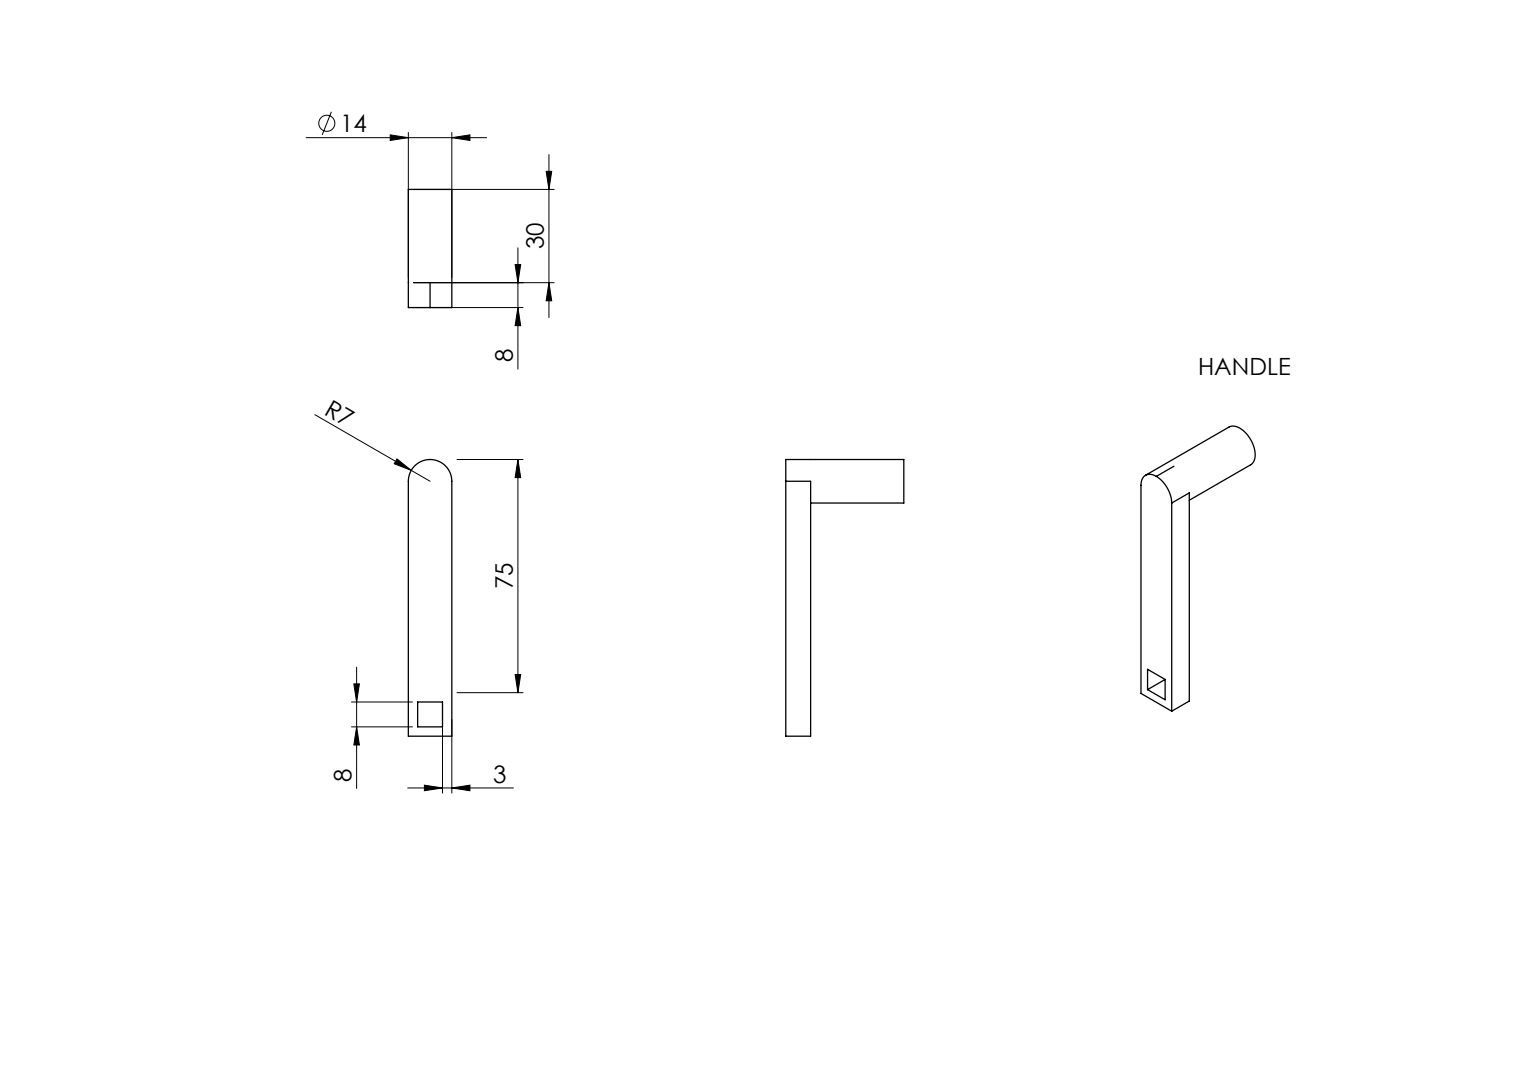
ISO-10303-21;
HEADER;
FILE_DESCRIPTION (('STEP AP214'),
    '1' );
FILE_NAME ('handle.step',
    '2026-10-27T17:01:19',
    ( '' ),
    ( '' ),
    'SwSTEP 2.0',
    'SolidWorks 2026',
    '' );
FILE_SCHEMA (( 'AUTOMOTIVE_DESIGN' ));
ENDSEC;

DATA;
#44=DIRECTION ( 'NONE',  ( 1.000000000000000000, 0.000000000000000000, -0.000000000000000000 ) ) ;
#60=PLANE ( 'NONE',  #2621 ) ;
#78=DIRECTION ( 'NONE',  ( 0.000000000000000000, 0.000000000000000000, -1.000000000000000000 ) ) ;
#181=DIRECTION ( 'NONE',  ( 1.000000000000000000, 0.000000000000000000, 0.000000000000000000 ) ) ;
#209=FACE_OUTER_BOUND ( 'NONE', #12548, .T. ) ;
#242=EDGE_CURVE ( 'NONE', #7278, #11617, #2972, .T. ) ;
#243=ADVANCED_FACE ( 'NONE', ( #12113 ), #8583, .F. ) ;
#284=UNCERTAINTY_MEASURE_WITH_UNIT (LENGTH_MEASURE( 1.000000000000000082E-05 ), #8450, 'distance_accuracy_value', 'NONE');
#293=VERTEX_POINT ( 'NONE', #4374 ) ;
#306=ORIENTED_EDGE ( 'NONE', *, *, #7465, .F. ) ;
#327=ORIENTED_EDGE ( 'NONE', *, *, #242, .F. ) ;
#406=CIRCLE ( 'NONE', #2294, 7.000000000000006217 ) ;
#523=EDGE_CURVE ( 'NONE', #5999, #556, #4821, .T. ) ;
#539=ORIENTED_EDGE ( 'NONE', *, *, #671, .F. ) ;
#556=VERTEX_POINT ( 'NONE', #3859 ) ;
#601=CARTESIAN_POINT ( 'NONE',  ( 639.0000000000000000, 164.0000000000000000, -225.5000000000000000 ) ) ;
#617=EDGE_CURVE ( 'NONE', #4863, #2268, #5468, .T. ) ;
#643=CIRCLE ( 'NONE', #14334, 7.000000000000006217 ) ;
#671=EDGE_CURVE ( 'NONE', #9854, #4863, #4289, .T. ) ;
#696=VERTEX_POINT ( 'NONE', #14184 ) ;
#712=CARTESIAN_POINT ( 'NONE',  ( 642.0000000000000000, 235.0000000000000284, -263.5000000000000000 ) ) ;
#748=SHAPE_REPRESENTATION ( 'handle', ( #9440 ), #10411 ) ;
#775=( NAMED_UNIT ( * ) PLANE_ANGLE_UNIT ( ) SI_UNIT ( $, .RADIAN. ) );
#845=ORIENTED_EDGE ( 'NONE', *, *, #1115, .T. ) ;
#886=DIRECTION ( 'NONE',  ( 0.000000000000000000, -1.000000000000000000, 0.000000000000000000 ) ) ;
#911=( NAMED_UNIT ( * ) SI_UNIT ( $, .STERADIAN. ) SOLID_ANGLE_UNIT ( ) );
#1008=AXIS2_PLACEMENT_3D ( 'NONE', #14417, #7766, #13089 ) ;
#1086=CARTESIAN_POINT ( 'NONE',  ( 635.0000000000000000, 235.0000000000000284, -233.5000000000000000 ) ) ;
#1115=EDGE_CURVE ( 'NONE', #10699, #12031, #8189, .T. ) ;
#1162=FACE_OUTER_BOUND ( 'NONE', #3028, .T. ) ;
#1261=FACE_OUTER_BOUND ( 'NONE', #8689, .T. ) ;
#1269=ORIENTED_EDGE ( 'NONE', *, *, #6620, .T. ) ;
#1282=EDGE_LOOP ( 'NONE', ( #8949, #7647, #11738, #7924 ) ) ;
#1314=CYLINDRICAL_SURFACE ( 'NONE', #12760, 7.000000000000006217 ) ;
#1346=AXIS2_PLACEMENT_3D ( 'NONE', #14026, #11711, #4877 ) ;
#1349=ORIENTED_EDGE ( 'NONE', *, *, #7002, .F. ) ;
#1361=VECTOR ( 'NONE', #4691, 1000.000000000000000 ) ;
#1453=STYLED_ITEM ( 'NONE', ( #1805 ), #3692 ) ;
#1476=PRODUCT_DEFINITION_FORMATION_WITH_SPECIFIED_SOURCE ( 'ANY', '', #5136, .NOT_KNOWN. ) ;
#1478=FACE_OUTER_BOUND ( 'NONE', #1563, .T. ) ;
#1563=EDGE_LOOP ( 'NONE', ( #9615, #3354, #5095, #1269 ) ) ;
#1583=ORIENTED_EDGE ( 'NONE', *, *, #617, .F. ) ;
#1626=DIRECTION ( 'NONE',  ( 1.000000000000000000, -3.469446951953611033E-15, 0.000000000000000000 ) ) ;
#1713=ADVANCED_FACE ( 'NONE', ( #209 ), #4604, .T. ) ;
#1799=CARTESIAN_POINT ( 'NONE',  ( 631.0000000000000000, 155.9999999999999432, -233.5000000000000000 ) ) ;
#1805=PRESENTATION_STYLE_ASSIGNMENT (( #2092 ) ) ;
#1807=( NAMED_UNIT ( * ) SI_UNIT ( $, .STERADIAN. ) SOLID_ANGLE_UNIT ( ) );
#1893=LINE ( 'NONE', #2781, #8946 ) ;
#1921=CARTESIAN_POINT ( 'NONE',  ( 639.0000000000000000, 164.0000000000000000, -233.5000000000000000 ) ) ;
#1968=ORIENTED_EDGE ( 'NONE', *, *, #9334, .T. ) ;
#2004=CARTESIAN_POINT ( 'NONE',  ( 628.0000000000000000, 235.0000000000000284, -225.5000000000000000 ) ) ;
#2020=SURFACE_SIDE_STYLE ('',( #2931 ) ) ;
#2039=ORIENTED_EDGE ( 'NONE', *, *, #6133, .F. ) ;
#2046=VECTOR ( 'NONE', #12296, 1000.000000000000000 ) ;
#2070=LINE ( 'NONE', #9225, #10344 ) ;
#2088=VECTOR ( 'NONE', #3181, 1000.000000000000000 ) ;
#2092=SURFACE_STYLE_USAGE ( .BOTH. , #2020 ) ;
#2195=ADVANCED_FACE ( 'NONE', ( #1478 ), #10477, .F. ) ;
#2246=APPLICATION_CONTEXT ( 'automotive_design' ) ;
#2268=VERTEX_POINT ( 'NONE', #1799 ) ;
#2294=AXIS2_PLACEMENT_3D ( 'NONE', #14046, #7317, #14110 ) ;
#2329=VECTOR ( 'NONE', #2494, 1000.000000000000000 ) ;
#2412=EDGE_CURVE ( 'NONE', #7278, #12527, #643, .T. ) ;
#2425=EDGE_CURVE ( 'NONE', #293, #556, #406, .T. ) ;
#2439=CLOSED_SHELL ( 'NONE', ( #8354, #13277, #14507, #10352, #2195, #243, #12766, #10082, #1713, #5998, #10469, #5380 ) ) ;
#2494=DIRECTION ( 'NONE',  ( 0.000000000000000000, 0.000000000000000000, 1.000000000000000000 ) ) ;
#2621=AXIS2_PLACEMENT_3D ( 'NONE', #4525, #4597, #3477 ) ;
#2651=CARTESIAN_POINT ( 'NONE',  ( 642.0000000000000000, 153.0000000000000284, -225.5000000000000000 ) ) ;
#2671=VERTEX_POINT ( 'NONE', #13959 ) ;
#2734=LINE ( 'NONE', #11726, #9172 ) ;
#2781=CARTESIAN_POINT ( 'NONE',  ( 639.0000000000000000, 164.0000000000000000, -233.5000000000000000 ) ) ;
#2842=AXIS2_PLACEMENT_3D ( 'NONE', #3398, #7894, #44 ) ;
#2908=DIRECTION ( 'NONE',  ( 1.000000000000000000, 0.000000000000000000, -0.000000000000000000 ) ) ;
#2923=CARTESIAN_POINT ( 'NONE',  ( 631.0000000000000000, 164.0000000000000284, -233.5000000000000000 ) ) ;
#2931=SURFACE_STYLE_FILL_AREA ( #12136 ) ;
#2972=LINE ( 'NONE', #9832, #5262 ) ;
#3028=EDGE_LOOP ( 'NONE', ( #5579, #7466, #3469, #11581 ) ) ;
#3157=DIRECTION ( 'NONE',  ( -0.000000000000000000, -0.000000000000000000, 1.000000000000000000 ) ) ;
#3181=DIRECTION ( 'NONE',  ( -1.000000000000000000, -7.930164461608254918E-15, 0.000000000000000000 ) ) ;
#3213=( NAMED_UNIT ( * ) PLANE_ANGLE_UNIT ( ) SI_UNIT ( $, .RADIAN. ) );
#3251=ORIENTED_EDGE ( 'NONE', *, *, #4308, .T. ) ;
#3320=FACE_OUTER_BOUND ( 'NONE', #1282, .T. ) ;
#3354=ORIENTED_EDGE ( 'NONE', *, *, #8629, .F. ) ;
#3398=CARTESIAN_POINT ( 'NONE',  ( 0.000000000000000000, 0.000000000000000000, -225.5000000000000000 ) ) ;
#3430=VERTEX_POINT ( 'NONE', #11452 ) ;
#3469=ORIENTED_EDGE ( 'NONE', *, *, #6926, .T. ) ;
#3477=DIRECTION ( 'NONE',  ( -1.000000000000000000, -6.938893903907222067E-15, 0.000000000000000000 ) ) ;
#3534=VECTOR ( 'NONE', #13559, 1000.000000000000000 ) ;
#3558=AXIS2_PLACEMENT_3D ( 'NONE', #6429, #10928, #13211 ) ;
#3631=ORIENTED_EDGE ( 'NONE', *, *, #4308, .F. ) ;
#3642=DIRECTION ( 'NONE',  ( -1.000000000000000000, 0.000000000000000000, -0.000000000000000000 ) ) ;
#3653=ORIENTED_EDGE ( 'NONE', *, *, #2412, .T. ) ;
#3692=ADVANCED_BREP_SHAPE_REPRESENTATION ( '', ( #7462, #9440 ), #10411 ) ;
#3695=DIRECTION ( 'NONE',  ( -0.000000000000000000, 1.000000000000000000, -0.000000000000000000 ) ) ;
#3726=CARTESIAN_POINT ( 'NONE',  ( 635.0000000000000000, 235.0000000000000284, -263.5000000000000000 ) ) ;
#3785=VECTOR ( 'NONE', #11447, 1000.000000000000000 ) ;
#3802=DIRECTION ( 'NONE',  ( 0.000000000000000000, -0.000000000000000000, 1.000000000000000000 ) ) ;
#3859=CARTESIAN_POINT ( 'NONE',  ( 628.0000000000000000, 235.0000000000000284, -233.5000000000000000 ) ) ;
#3979=ORIENTED_EDGE ( 'NONE', *, *, #13006, .T. ) ;
#4038=VECTOR ( 'NONE', #3157, 1000.000000000000000 ) ;
#4076=DIRECTION ( 'NONE',  ( 0.000000000000000000, -1.000000000000000000, 0.000000000000000000 ) ) ;
#4133=ORIENTED_EDGE ( 'NONE', *, *, #7825, .T. ) ;
#4140=PLANE ( 'NONE',  #3558 ) ;
#4188=EDGE_LOOP ( 'NONE', ( #10021, #13008, #3979, #8499 ) ) ;
#4260=LINE ( 'NONE', #13265, #4038 ) ;
#4289=LINE ( 'NONE', #1921, #9835 ) ;
#4308=EDGE_CURVE ( 'NONE', #9854, #4571, #1893, .T. ) ;
#4317=EDGE_LOOP ( 'NONE', ( #845, #4133 ) ) ;
#4347=CARTESIAN_POINT ( 'NONE',  ( 0.000000000000000000, 0.000000000000000000, 0.000000000000000000 ) ) ;
#4361=CARTESIAN_POINT ( 'NONE',  ( 639.0000000000000000, 156.0000000000000000, -233.5000000000000000 ) ) ;
#4374=CARTESIAN_POINT ( 'NONE',  ( 642.0000000000000000, 235.0000000000000284, -233.5000000000000000 ) ) ;
#4395=PRODUCT_DEFINITION_SHAPE ( 'NONE', 'NONE',  #9740 ) ;
#4525=CARTESIAN_POINT ( 'NONE',  ( 639.0000000000000000, 156.0000000000000000, -233.5000000000000000 ) ) ;
#4571=VERTEX_POINT ( 'NONE', #9274 ) ;
#4597=DIRECTION ( 'NONE',  ( -6.938893903907222067E-15, 1.000000000000000000, 0.000000000000000000 ) ) ;
#4604=PLANE ( 'NONE',  #7505 ) ;
#4613=ORIENTED_EDGE ( 'NONE', *, *, #2412, .F. ) ;
#4643=DIRECTION ( 'NONE',  ( 0.000000000000000000, 0.000000000000000000, -1.000000000000000000 ) ) ;
#4649=DIRECTION ( 'NONE',  ( -0.000000000000000000, -0.000000000000000000, 1.000000000000000000 ) ) ;
#4691=DIRECTION ( 'NONE',  ( -0.000000000000000000, -0.000000000000000000, 1.000000000000000000 ) ) ;
#4715=CARTESIAN_POINT ( 'NONE',  ( 642.0000000000000000, 235.0000000000000284, -225.5000000000000000 ) ) ;
#4756=CARTESIAN_POINT ( 'NONE',  ( 631.0000000000000000, 155.9999999999999432, -233.5000000000000000 ) ) ;
#4757=CARTESIAN_POINT ( 'NONE',  ( 639.0000000000000000, 164.0000000000000000, -233.5000000000000000 ) ) ;
#4799=EDGE_LOOP ( 'NONE', ( #539, #13382, #5109, #1583 ) ) ;
#4802=PLANE ( 'NONE',  #11798 ) ;
#4821=LINE ( 'NONE', #9381, #6730 ) ;
#4863=VERTEX_POINT ( 'NONE', #5346 ) ;
#4877=DIRECTION ( 'NONE',  ( -1.000000000000000000, -7.930164461608254918E-15, 0.000000000000000000 ) ) ;
#4886=UNCERTAINTY_MEASURE_WITH_UNIT (LENGTH_MEASURE( 1.000000000000000082E-05 ), #12067, 'distance_accuracy_value', 'NONE');
#5001=VECTOR ( 'NONE', #6147, 1000.000000000000000 ) ;
#5029=ORIENTED_EDGE ( 'NONE', *, *, #8532, .F. ) ;
#5070=CARTESIAN_POINT ( 'NONE',  ( 631.0000000000000000, 155.9999999999999432, -233.5000000000000000 ) ) ;
#5072=DIRECTION ( 'NONE',  ( 0.000000000000000000, 0.000000000000000000, 1.000000000000000000 ) ) ;
#5095=ORIENTED_EDGE ( 'NONE', *, *, #13006, .F. ) ;
#5109=ORIENTED_EDGE ( 'NONE', *, *, #8864, .F. ) ;
#5136=PRODUCT ( 'handle', 'handle', '', ( #12319 ) ) ;
#5210=DIRECTION ( 'NONE',  ( -3.469446951953611033E-15, -1.000000000000000000, 0.000000000000000000 ) ) ;
#5262=VECTOR ( 'NONE', #886, 1000.000000000000000 ) ;
#5346=CARTESIAN_POINT ( 'NONE',  ( 639.0000000000000000, 156.0000000000000000, -233.5000000000000000 ) ) ;
#5380=ADVANCED_FACE ( 'NONE', ( #8162 ), #4802, .T. ) ;
#5411=LINE ( 'NONE', #8735, #13411 ) ;
#5468=LINE ( 'NONE', #4361, #10058 ) ;
#5472=SHAPE_DEFINITION_REPRESENTATION ( #4395, #748 ) ;
#5482=CARTESIAN_POINT ( 'NONE',  ( 639.0000000000000000, 164.0000000000000000, -233.5000000000000000 ) ) ;
#5511=( NAMED_UNIT ( * ) PLANE_ANGLE_UNIT ( ) SI_UNIT ( $, .RADIAN. ) );
#5522=ORIENTED_EDGE ( 'NONE', *, *, #8833, .F. ) ;
#5579=ORIENTED_EDGE ( 'NONE', *, *, #5949, .F. ) ;
#5660=CIRCLE ( 'NONE', #10848, 7.000000000000006217 ) ;
#5680=FACE_OUTER_BOUND ( 'NONE', #14377, .T. ) ;
#5698=FACE_OUTER_BOUND ( 'NONE', #11324, .T. ) ;
#5785=LINE ( 'NONE', #10287, #1361 ) ;
#5887=DIRECTION ( 'NONE',  ( 0.000000000000000000, 0.000000000000000000, 1.000000000000000000 ) ) ;
#5949=EDGE_CURVE ( 'NONE', #12031, #556, #6306, .T. ) ;
#5998=ADVANCED_FACE ( 'NONE', ( #9635 ), #13036, .T. ) ;
#5999=VERTEX_POINT ( 'NONE', #8375 ) ;
#6011=LINE ( 'NONE', #5070, #13941 ) ;
#6133=EDGE_CURVE ( 'NONE', #12527, #556, #8091, .T. ) ;
#6140=FACE_OUTER_BOUND ( 'NONE', #10952, .T. ) ;
#6147=DIRECTION ( 'NONE',  ( 0.000000000000000000, 1.000000000000000000, 0.000000000000000000 ) ) ;
#6306=LINE ( 'NONE', #10738, #12414 ) ;
#6316=( NAMED_UNIT ( * ) SI_UNIT ( $, .STERADIAN. ) SOLID_ANGLE_UNIT ( ) );
#6319=DIRECTION ( 'NONE',  ( -1.000000000000000000, -6.938893903907222067E-15, 0.000000000000000000 ) ) ;
#6366=CARTESIAN_POINT ( 'NONE',  ( 642.0000000000000000, 153.0000000000000284, -233.5000000000000000 ) ) ;
#6411=DIRECTION ( 'NONE',  ( -0.000000000000000000, -0.000000000000000000, 1.000000000000000000 ) ) ;
#6417=DIRECTION ( 'NONE',  ( 1.000000000000000000, 0.000000000000000000, 0.000000000000000000 ) ) ;
#6429=CARTESIAN_POINT ( 'NONE',  ( 642.0000000000000000, 167.0000000000000000, -233.5000000000000000 ) ) ;
#6461=ORIENTED_EDGE ( 'NONE', *, *, #9334, .F. ) ;
#6476=ORIENTED_EDGE ( 'NONE', *, *, #7002, .T. ) ;
#6620=EDGE_CURVE ( 'NONE', #13306, #11617, #5785, .T. ) ;
#6665=UNCERTAINTY_MEASURE_WITH_UNIT (LENGTH_MEASURE( 1.000000000000000082E-05 ), #8676, 'distance_accuracy_value', 'NONE');
#6730=VECTOR ( 'NONE', #12697, 1000.000000000000000 ) ;
#6777=APPLICATION_CONTEXT ( 'automotive_design' ) ;
#6827=VECTOR ( 'NONE', #8383, 1000.000000000000000 ) ;
#6914=EDGE_CURVE ( 'NONE', #11617, #2671, #5411, .T. ) ;
#6926=EDGE_CURVE ( 'NONE', #10699, #293, #9985, .T. ) ;
#6952=LINE ( 'NONE', #13372, #3785 ) ;
#7002=EDGE_CURVE ( 'NONE', #4863, #13301, #2070, .T. ) ;
#7072=CARTESIAN_POINT ( 'NONE',  ( 642.0000000000000000, 235.0000000000000284, -233.5000000000000000 ) ) ;
#7103=LINE ( 'NONE', #9393, #5001 ) ;
#7199=DIRECTION ( 'NONE',  ( 1.000000000000000000, -3.469446951953611033E-15, 0.000000000000000000 ) ) ;
#7262=ORIENTED_EDGE ( 'NONE', *, *, #13827, .F. ) ;
#7278=VERTEX_POINT ( 'NONE', #4715 ) ;
#7283=EDGE_CURVE ( 'NONE', #9217, #9854, #13628, .T. ) ;
#7317=DIRECTION ( 'NONE',  ( 0.000000000000000000, 0.000000000000000000, -1.000000000000000000 ) ) ;
#7410=EDGE_CURVE ( 'NONE', #2268, #696, #10463, .T. ) ;
#7462=MANIFOLD_SOLID_BREP ( 'Boss-Extrude2', #2439 ) ;
#7465=EDGE_CURVE ( 'NONE', #13301, #696, #12200, .T. ) ;
#7466=ORIENTED_EDGE ( 'NONE', *, *, #1115, .F. ) ;
#7475=DIRECTION ( 'NONE',  ( -1.000000000000000000, -7.930164461608254918E-15, 0.000000000000000000 ) ) ;
#7505=AXIS2_PLACEMENT_3D ( 'NONE', #4756, #9244, #9091 ) ;
#7612=ORIENTED_EDGE ( 'NONE', *, *, #7410, .F. ) ;
#7647=ORIENTED_EDGE ( 'NONE', *, *, #13827, .T. ) ;
#7766=DIRECTION ( 'NONE',  ( 1.000000000000000000, 0.000000000000000000, 0.000000000000000000 ) ) ;
#7768=MECHANICAL_DESIGN_GEOMETRIC_PRESENTATION_REPRESENTATION('',(#11527),#12714);
#7825=EDGE_CURVE ( 'NONE', #12031, #10699, #5660, .T. ) ;
#7887=EDGE_CURVE ( 'NONE', #293, #13306, #6952, .T. ) ;
#7894=DIRECTION ( 'NONE',  ( 0.000000000000000000, -0.000000000000000000, 1.000000000000000000 ) ) ;
#7924=ORIENTED_EDGE ( 'NONE', *, *, #6620, .F. ) ;
#7981=ORIENTED_EDGE ( 'NONE', *, *, #8532, .T. ) ;
#8040=VECTOR ( 'NONE', #10369, 1000.000000000000000 ) ;
#8091=LINE ( 'NONE', #10235, #2046 ) ;
#8122=DIRECTION ( 'NONE',  ( -0.000000000000000000, 0.000000000000000000, 1.000000000000000000 ) ) ;
#8162=FACE_OUTER_BOUND ( 'NONE', #4317, .T. ) ;
#8189=CIRCLE ( 'NONE', #13624, 7.000000000000006217 ) ;
#8202=AXIS2_PLACEMENT_3D ( 'NONE', #4757, #3642, #8122 ) ;
#8234=VECTOR ( 'NONE', #6319, 1000.000000000000000 ) ;
#8306=ORIENTED_EDGE ( 'NONE', *, *, #7825, .F. ) ;
#8354=ADVANCED_FACE ( 'NONE', ( #1261 ), #11147, .T. ) ;
#8375=CARTESIAN_POINT ( 'NONE',  ( 628.0000000000000000, 152.9999999999999147, -233.5000000000000000 ) ) ;
#8383=DIRECTION ( 'NONE',  ( -0.000000000000000000, -0.000000000000000000, 1.000000000000000000 ) ) ;
#8385=ORIENTED_EDGE ( 'NONE', *, *, #5949, .T. ) ;
#8450=( LENGTH_UNIT ( ) NAMED_UNIT ( * ) SI_UNIT ( .MILLI., .METRE. ) );
#8499=ORIENTED_EDGE ( 'NONE', *, *, #523, .T. ) ;
#8532=EDGE_CURVE ( 'NONE', #2671, #12527, #9231, .T. ) ;
#8583=PLANE ( 'NONE',  #1008 ) ;
#8591=CARTESIAN_POINT ( 'NONE',  ( 635.0000000000000000, 235.0000000000000284, -263.5000000000000000 ) ) ;
#8629=EDGE_CURVE ( 'NONE', #5999, #2671, #4260, .T. ) ;
#8676=( LENGTH_UNIT ( ) NAMED_UNIT ( * ) SI_UNIT ( .MILLI., .METRE. ) );
#8689=EDGE_LOOP ( 'NONE', ( #8306, #8385, #2039, #4613, #7262, #10315 ) ) ;
#8722=VECTOR ( 'NONE', #14008, 1000.000000000000000 ) ;
#8735=CARTESIAN_POINT ( 'NONE',  ( 642.0000000000000000, 153.0000000000000284, -225.5000000000000000 ) ) ;
#8759=SHAPE_REPRESENTATION_RELATIONSHIP ( 'NONE' , 'NONE' ,  #748, #3692 ) ;
#8808=DIRECTION ( 'NONE',  ( 0.000000000000000000, -1.000000000000000000, 0.000000000000000000 ) ) ;
#8833=EDGE_CURVE ( 'NONE', #9217, #3430, #12358, .T. ) ;
#8864=EDGE_CURVE ( 'NONE', #2268, #9217, #6011, .T. ) ;
#8928=CARTESIAN_POINT ( 'NONE',  ( 642.0000000000000000, 153.0000000000000284, -233.5000000000000000 ) ) ;
#8946=VECTOR ( 'NONE', #6411, 1000.000000000000000 ) ;
#8949=ORIENTED_EDGE ( 'NONE', *, *, #7887, .F. ) ;
#9002=PLANE ( 'NONE',  #2842 ) ;
#9078=DIRECTION ( 'NONE',  ( 0.000000000000000000, 0.000000000000000000, 1.000000000000000000 ) ) ;
#9091=DIRECTION ( 'NONE',  ( 0.000000000000000000, 0.000000000000000000, -1.000000000000000000 ) ) ;
#9126=AXIS2_PLACEMENT_3D ( 'NONE', #2923, #5210, #7199 ) ;
#9172=VECTOR ( 'NONE', #1626, 1000.000000000000000 ) ;
#9210=EDGE_LOOP ( 'NONE', ( #13436, #5522, #12148, #3251 ) ) ;
#9217=VERTEX_POINT ( 'NONE', #10051 ) ;
#9225=CARTESIAN_POINT ( 'NONE',  ( 639.0000000000000000, 156.0000000000000000, -233.5000000000000000 ) ) ;
#9231=LINE ( 'NONE', #12547, #11564 ) ;
#9232=( GEOMETRIC_REPRESENTATION_CONTEXT ( 3 ) GLOBAL_UNCERTAINTY_ASSIGNED_CONTEXT ( ( #4886 ) ) GLOBAL_UNIT_ASSIGNED_CONTEXT ( ( #12067, #775, #6316 ) ) REPRESENTATION_CONTEXT ( 'NONE', 'WORKASPACE' ) );
#9244=DIRECTION ( 'NONE',  ( 1.000000000000000000, -0.000000000000000000, 0.000000000000000000 ) ) ;
#9274=CARTESIAN_POINT ( 'NONE',  ( 639.0000000000000000, 164.0000000000000000, -225.5000000000000000 ) ) ;
#9316=PLANE ( 'NONE',  #8202 ) ;
#9334=EDGE_CURVE ( 'NONE', #696, #3430, #7103, .T. ) ;
#9381=CARTESIAN_POINT ( 'NONE',  ( 628.0000000000000000, 152.9999999999999147, -233.5000000000000000 ) ) ;
#9393=CARTESIAN_POINT ( 'NONE',  ( 631.0000000000000000, 155.9999999999999432, -225.5000000000000000 ) ) ;
#9440=AXIS2_PLACEMENT_3D ( 'NONE', #4347, #14302, #6417 ) ;
#9544=DIRECTION ( 'NONE',  ( 1.000000000000000000, 0.000000000000000000, 0.000000000000000000 ) ) ;
#9613=CARTESIAN_POINT ( 'NONE',  ( 0.000000000000000000, 0.000000000000000000, -233.5000000000000000 ) ) ;
#9615=ORIENTED_EDGE ( 'NONE', *, *, #6914, .T. ) ;
#9635=FACE_OUTER_BOUND ( 'NONE', #9210, .T. ) ;
#9655=AXIS2_PLACEMENT_3D ( 'NONE', #9613, #3802, #2908 ) ;
#9696=FACE_BOUND ( 'NONE', #4799, .T. ) ;
#9740=PRODUCT_DEFINITION ( 'UNKNOWN', '', #1476, #13744 ) ;
#9826=DIRECTION ( 'NONE',  ( 0.000000000000000000, -0.000000000000000000, 1.000000000000000000 ) ) ;
#9832=CARTESIAN_POINT ( 'NONE',  ( 642.0000000000000000, 167.0000000000000000, -225.5000000000000000 ) ) ;
#9835=VECTOR ( 'NONE', #4076, 1000.000000000000000 ) ;
#9854=VERTEX_POINT ( 'NONE', #5482 ) ;
#9985=LINE ( 'NONE', #7072, #2329 ) ;
#10021=ORIENTED_EDGE ( 'NONE', *, *, #2425, .F. ) ;
#10051=CARTESIAN_POINT ( 'NONE',  ( 631.0000000000000000, 164.0000000000000284, -233.5000000000000000 ) ) ;
#10058=VECTOR ( 'NONE', #14254, 1000.000000000000000 ) ;
#10082=ADVANCED_FACE ( 'NONE', ( #5698 ), #60, .T. ) ;
#10102=FACE_BOUND ( 'NONE', #11103, .T. ) ;
#10223=ORIENTED_EDGE ( 'NONE', *, *, #671, .T. ) ;
#10235=CARTESIAN_POINT ( 'NONE',  ( 628.0000000000000000, 235.0000000000000284, -233.5000000000000000 ) ) ;
#10268=ORIENTED_EDGE ( 'NONE', *, *, #8629, .T. ) ;
#10287=CARTESIAN_POINT ( 'NONE',  ( 642.0000000000000000, 153.0000000000000284, -233.5000000000000000 ) ) ;
#10315=ORIENTED_EDGE ( 'NONE', *, *, #6926, .F. ) ;
#10344=VECTOR ( 'NONE', #4649, 1000.000000000000000 ) ;
#10352=ADVANCED_FACE ( 'NONE', ( #3320 ), #4140, .F. ) ;
#10369=DIRECTION ( 'NONE',  ( -0.000000000000000000, -0.000000000000000000, 1.000000000000000000 ) ) ;
#10411=( GEOMETRIC_REPRESENTATION_CONTEXT ( 3 ) GLOBAL_UNCERTAINTY_ASSIGNED_CONTEXT ( ( #284 ) ) GLOBAL_UNIT_ASSIGNED_CONTEXT ( ( #8450, #3213, #911 ) ) REPRESENTATION_CONTEXT ( 'NONE', 'WORKASPACE' ) );
#10463=LINE ( 'NONE', #14012, #6827 ) ;
#10468=CARTESIAN_POINT ( 'NONE',  ( 635.0000000000000000, 235.0000000000000284, -263.5000000000000000 ) ) ;
#10469=ADVANCED_FACE ( 'NONE', ( #1162 ), #1314, .T. ) ;
#10477=PLANE ( 'NONE',  #1346 ) ;
#10569=VECTOR ( 'NONE', #8808, 1000.000000000000000 ) ;
#10653=FACE_OUTER_BOUND ( 'NONE', #4188, .T. ) ;
#10699=VERTEX_POINT ( 'NONE', #712 ) ;
#10723=ORIENTED_EDGE ( 'NONE', *, *, #12824, .T. ) ;
#10738=CARTESIAN_POINT ( 'NONE',  ( 628.0000000000000000, 235.0000000000000284, -233.5000000000000000 ) ) ;
#10758=ORIENTED_EDGE ( 'NONE', *, *, #523, .F. ) ;
#10848=AXIS2_PLACEMENT_3D ( 'NONE', #8591, #14127, #12184 ) ;
#10928=DIRECTION ( 'NONE',  ( -1.000000000000000000, 0.000000000000000000, -0.000000000000000000 ) ) ;
#10947=LINE ( 'NONE', #601, #10569 ) ;
#10952=EDGE_LOOP ( 'NONE', ( #12806, #3631, #10223, #6476 ) ) ;
#11103=EDGE_LOOP ( 'NONE', ( #10723, #12617, #13595, #1968 ) ) ;
#11147=CYLINDRICAL_SURFACE ( 'NONE', #14395, 7.000000000000006217 ) ;
#11215=DIRECTION ( 'NONE',  ( 1.000000000000000000, 0.000000000000000000, 0.000000000000000000 ) ) ;
#11216=ORIENTED_EDGE ( 'NONE', *, *, #6133, .T. ) ;
#11324=EDGE_LOOP ( 'NONE', ( #306, #1349, #12354, #12390 ) ) ;
#11447=DIRECTION ( 'NONE',  ( -0.000000000000000000, -1.000000000000000000, -0.000000000000000000 ) ) ;
#11452=CARTESIAN_POINT ( 'NONE',  ( 631.0000000000000000, 164.0000000000000284, -225.5000000000000000 ) ) ;
#11527=STYLED_ITEM('',(#14667),#7462);
#11564=VECTOR ( 'NONE', #3695, 1000.000000000000000 ) ;
#11581=ORIENTED_EDGE ( 'NONE', *, *, #2425, .T. ) ;
#11607=EDGE_LOOP ( 'NONE', ( #7981, #11216, #10758, #10268 ) ) ;
#11617=VERTEX_POINT ( 'NONE', #2651 ) ;
#11629=CARTESIAN_POINT ( 'NONE',  ( 642.0000000000000000, 235.0000000000000284, -233.5000000000000000 ) ) ;
#11711=DIRECTION ( 'NONE',  ( -7.930164461608254918E-15, 1.000000000000000000, 0.000000000000000000 ) ) ;
#11726=CARTESIAN_POINT ( 'NONE',  ( 631.0000000000000000, 164.0000000000000284, -225.5000000000000000 ) ) ;
#11737=CARTESIAN_POINT ( 'NONE',  ( 639.0000000000000000, 156.0000000000000000, -225.5000000000000000 ) ) ;
#11738=ORIENTED_EDGE ( 'NONE', *, *, #242, .T. ) ;
#11754=DIRECTION ( 'NONE',  ( 0.000000000000000000, 1.000000000000000000, 0.000000000000000000 ) ) ;
#11798=AXIS2_PLACEMENT_3D ( 'NONE', #10468, #4643, #13944 ) ;
#12031=VERTEX_POINT ( 'NONE', #13933 ) ;
#12067=( LENGTH_UNIT ( ) NAMED_UNIT ( * ) SI_UNIT ( .MILLI., .METRE. ) );
#12113=FACE_OUTER_BOUND ( 'NONE', #11607, .T. ) ;
#12136=FILL_AREA_STYLE ('',( #14223 ) ) ;
#12148=ORIENTED_EDGE ( 'NONE', *, *, #7283, .T. ) ;
#12184=DIRECTION ( 'NONE',  ( -1.000000000000000000, 0.000000000000000000, 0.000000000000000000 ) ) ;
#12200=LINE ( 'NONE', #14363, #8234 ) ;
#12296=DIRECTION ( 'NONE',  ( -0.000000000000000000, -0.000000000000000000, -1.000000000000000000 ) ) ;
#12319=PRODUCT_CONTEXT ( 'NONE', #6777, 'mechanical' ) ;
#12321=CARTESIAN_POINT ( 'NONE',  ( 635.0000000000000000, 235.0000000000000284, -233.5000000000000000 ) ) ;
#12354=ORIENTED_EDGE ( 'NONE', *, *, #617, .T. ) ;
#12358=LINE ( 'NONE', #13615, #8040 ) ;
#12386=LINE ( 'NONE', #8928, #2088 ) ;
#12390=ORIENTED_EDGE ( 'NONE', *, *, #7410, .T. ) ;
#12414=VECTOR ( 'NONE', #5072, 1000.000000000000000 ) ;
#12425=EDGE_CURVE ( 'NONE', #4571, #13301, #10947, .T. ) ;
#12527=VERTEX_POINT ( 'NONE', #2004 ) ;
#12547=CARTESIAN_POINT ( 'NONE',  ( 628.0000000000000000, 242.0000000000000568, -225.5000000000000000 ) ) ;
#12548=EDGE_LOOP ( 'NONE', ( #6461, #7612, #14130, #13391 ) ) ;
#12596=CARTESIAN_POINT ( 'NONE',  ( 631.0000000000000000, 164.0000000000000284, -233.5000000000000000 ) ) ;
#12617=ORIENTED_EDGE ( 'NONE', *, *, #12425, .T. ) ;
#12657=LINE ( 'NONE', #11629, #8722 ) ;
#12697=DIRECTION ( 'NONE',  ( 0.000000000000000000, 1.000000000000000000, 0.000000000000000000 ) ) ;
#12714=( GEOMETRIC_REPRESENTATION_CONTEXT ( 3 ) GLOBAL_UNCERTAINTY_ASSIGNED_CONTEXT ( ( #6665 ) ) GLOBAL_UNIT_ASSIGNED_CONTEXT ( ( #8676, #5511, #1807 ) ) REPRESENTATION_CONTEXT ( 'NONE', 'WORKASPACE' ) );
#12760=AXIS2_PLACEMENT_3D ( 'NONE', #1086, #5887, #181 ) ;
#12766=ADVANCED_FACE ( 'NONE', ( #6140 ), #9316, .T. ) ;
#12794=PLANE ( 'NONE',  #9655 ) ;
#12806=ORIENTED_EDGE ( 'NONE', *, *, #12425, .F. ) ;
#12824=EDGE_CURVE ( 'NONE', #3430, #4571, #2734, .T. ) ;
#13006=EDGE_CURVE ( 'NONE', #13306, #5999, #12386, .T. ) ;
#13008=ORIENTED_EDGE ( 'NONE', *, *, #7887, .T. ) ;
#13036=PLANE ( 'NONE',  #9126 ) ;
#13089=DIRECTION ( 'NONE',  ( 0.000000000000000000, 0.000000000000000000, -1.000000000000000000 ) ) ;
#13211=DIRECTION ( 'NONE',  ( -0.000000000000000000, 0.000000000000000000, 1.000000000000000000 ) ) ;
#13265=CARTESIAN_POINT ( 'NONE',  ( 628.0000000000000000, 152.9999999999999147, -233.5000000000000000 ) ) ;
#13277=ADVANCED_FACE ( 'NONE', ( #10653, #9696 ), #12794, .F. ) ;
#13301=VERTEX_POINT ( 'NONE', #11737 ) ;
#13306=VERTEX_POINT ( 'NONE', #6366 ) ;
#13372=CARTESIAN_POINT ( 'NONE',  ( 642.0000000000000000, 167.0000000000000000, -233.5000000000000000 ) ) ;
#13382=ORIENTED_EDGE ( 'NONE', *, *, #7283, .F. ) ;
#13391=ORIENTED_EDGE ( 'NONE', *, *, #8833, .T. ) ;
#13411=VECTOR ( 'NONE', #7475, 1000.000000000000000 ) ;
#13436=ORIENTED_EDGE ( 'NONE', *, *, #12824, .F. ) ;
#13476=MECHANICAL_DESIGN_GEOMETRIC_PRESENTATION_REPRESENTATION('',(#1453),#9232);
#13559=DIRECTION ( 'NONE',  ( 1.000000000000000000, -3.469446951953611033E-15, 0.000000000000000000 ) ) ;
#13595=ORIENTED_EDGE ( 'NONE', *, *, #7465, .T. ) ;
#13607=DIRECTION ( 'NONE',  ( -1.000000000000000000, 0.000000000000000000, 0.000000000000000000 ) ) ;
#13615=CARTESIAN_POINT ( 'NONE',  ( 631.0000000000000000, 164.0000000000000284, -233.5000000000000000 ) ) ;
#13624=AXIS2_PLACEMENT_3D ( 'NONE', #3726, #78, #13607 ) ;
#13628=LINE ( 'NONE', #12596, #3534 ) ;
#13710=COLOUR_RGB ( '',0.8941176470588234615, 0.8941176470588234615, 0.8941176470588234615 ) ;
#13744=PRODUCT_DEFINITION_CONTEXT ( 'detailed design', #2246, 'design' ) ;
#13747=ORIENTED_EDGE ( 'NONE', *, *, #6914, .F. ) ;
#13827=EDGE_CURVE ( 'NONE', #293, #7278, #12657, .T. ) ;
#13933=CARTESIAN_POINT ( 'NONE',  ( 628.0000000000000000, 235.0000000000000284, -263.5000000000000000 ) ) ;
#13941=VECTOR ( 'NONE', #11754, 1000.000000000000000 ) ;
#13944=DIRECTION ( 'NONE',  ( -1.000000000000000000, 0.000000000000000000, -0.000000000000000000 ) ) ;
#13959=CARTESIAN_POINT ( 'NONE',  ( 628.0000000000000000, 152.9999999999999147, -225.5000000000000000 ) ) ;
#14008=DIRECTION ( 'NONE',  ( 0.000000000000000000, 0.000000000000000000, 1.000000000000000000 ) ) ;
#14012=CARTESIAN_POINT ( 'NONE',  ( 631.0000000000000000, 155.9999999999999432, -233.5000000000000000 ) ) ;
#14026=CARTESIAN_POINT ( 'NONE',  ( 642.0000000000000000, 153.0000000000000284, -233.5000000000000000 ) ) ;
#14046=CARTESIAN_POINT ( 'NONE',  ( 635.0000000000000000, 235.0000000000000284, -233.5000000000000000 ) ) ;
#14110=DIRECTION ( 'NONE',  ( -1.000000000000000000, 0.000000000000000000, 0.000000000000000000 ) ) ;
#14127=DIRECTION ( 'NONE',  ( 0.000000000000000000, 0.000000000000000000, -1.000000000000000000 ) ) ;
#14130=ORIENTED_EDGE ( 'NONE', *, *, #8864, .T. ) ;
#14184=CARTESIAN_POINT ( 'NONE',  ( 631.0000000000000000, 155.9999999999999432, -225.5000000000000000 ) ) ;
#14223=FILL_AREA_STYLE_COLOUR ( '', #13710 ) ;
#14254=DIRECTION ( 'NONE',  ( -1.000000000000000000, -6.938893903907222067E-15, 0.000000000000000000 ) ) ;
#14262=CARTESIAN_POINT ( 'NONE',  ( 635.0000000000000000, 235.0000000000000284, -225.5000000000000000 ) ) ;
#14302=DIRECTION ( 'NONE',  ( 0.000000000000000000, 0.000000000000000000, 1.000000000000000000 ) ) ;
#14334=AXIS2_PLACEMENT_3D ( 'NONE', #14262, #9826, #9544 ) ;
#14363=CARTESIAN_POINT ( 'NONE',  ( 639.0000000000000000, 156.0000000000000000, -225.5000000000000000 ) ) ;
#14377=EDGE_LOOP ( 'NONE', ( #3653, #5029, #13747, #327 ) ) ;
#14395=AXIS2_PLACEMENT_3D ( 'NONE', #12321, #9078, #11215 ) ;
#14417=CARTESIAN_POINT ( 'NONE',  ( 628.0000000000000000, 242.0000000000000568, -233.5000000000000000 ) ) ;
#14507=ADVANCED_FACE ( 'NONE', ( #5680, #10102 ), #9002, .T. ) ;
#14661=COLOUR_RGB('Sky Blue',0.24,0.69,0.87);
#14662=FILL_AREA_STYLE_COLOUR('',#14661);
#14663=FILL_AREA_STYLE('',(#14662));
#14664=SURFACE_STYLE_FILL_AREA(#14663);
#14665=SURFACE_SIDE_STYLE('',(#14664));
#14666=SURFACE_STYLE_USAGE(.BOTH.,#14665);
#14667=PRESENTATION_STYLE_ASSIGNMENT((#14666));
ENDSEC;
END-ISO-10303-21;
